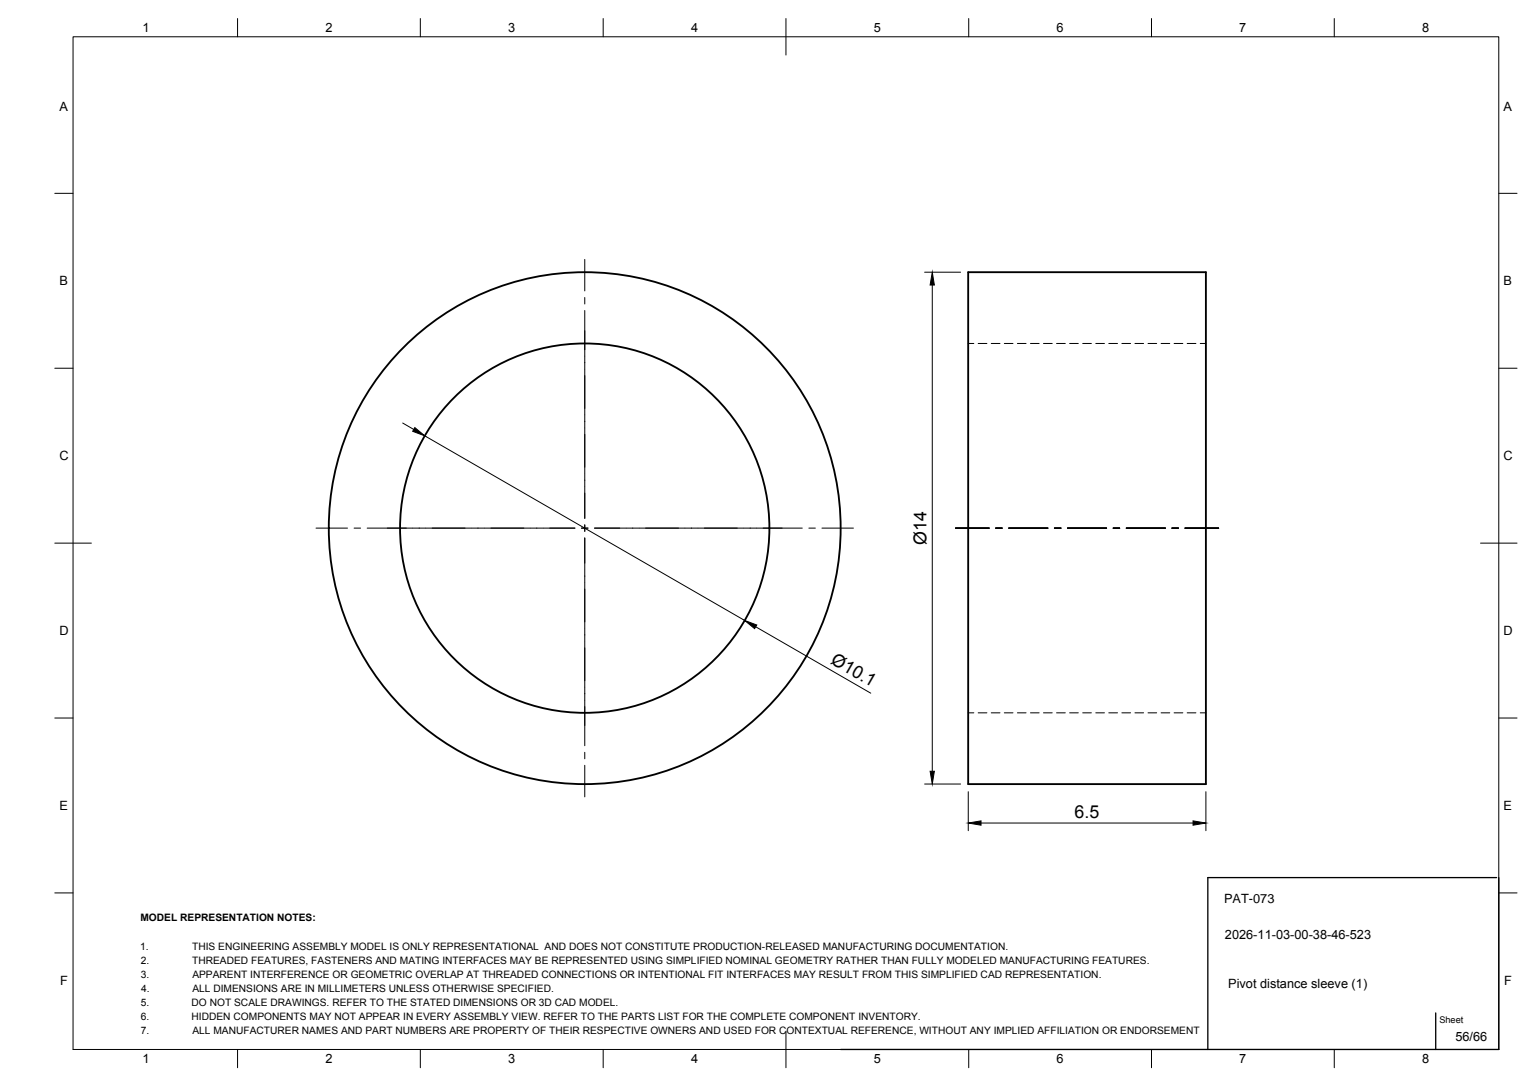
ISO-10303-21;
HEADER;
/* Generated by software containing ST-Developer
 * from STEP Tools, Inc. (www.steptools.com) 
 */

FILE_DESCRIPTION(
/* description */ ('Manual piston pump'),
/* implementation_level */ '2;1');

FILE_NAME(
/* name */ 'Pivot distance sleeve (1).step',
/* time_stamp */ '2026-11-02T16:54:23-08:00',
/* author */ (''),
/* organization */ (''),
/* preprocessor_version */ 'ST-DEVELOPER v20.2',
/* originating_system */ 'Autodesk Translation Framework v15.17.0.0',
/* authorisation */ '');

FILE_SCHEMA (('AUTOMOTIVE_DESIGN { 1 0 10303 214 3 1 1 }'));
ENDSEC;

DATA;
#10=MECHANICAL_DESIGN_GEOMETRIC_PRESENTATION_REPRESENTATION('',(#746),#19043);
#612=SHAPE_REPRESENTATION_RELATIONSHIP('SRR','None',#19362,#675);
#675=ADVANCED_BREP_SHAPE_REPRESENTATION('',(#814),#19029);
#746=STYLED_ITEM('',(#19664),#814);
#814=MANIFOLD_SOLID_BREP('Body1',#9534);
#1022=FACE_BOUND('',#2543,.T.);
#1023=FACE_BOUND('',#2545,.T.);
#1259=CYLINDRICAL_SURFACE('',#11283,0.505000000000001);
#1260=CYLINDRICAL_SURFACE('',#11286,0.699999999999999);
#1770=FACE_OUTER_BOUND('',#2540,.T.);
#1771=FACE_OUTER_BOUND('',#2541,.T.);
#1772=FACE_OUTER_BOUND('',#2542,.T.);
#1773=FACE_OUTER_BOUND('',#2544,.T.);
#2540=EDGE_LOOP('',(#8185,#8186,#8187,#8188));
#2541=EDGE_LOOP('',(#8189,#8190,#8191,#8192));
#2542=EDGE_LOOP('',(#8193));
#2543=EDGE_LOOP('',(#8194));
#2544=EDGE_LOOP('',(#8195));
#2545=EDGE_LOOP('',(#8196));
#3076=CIRCLE('',#11284,0.505000000000001);
#3077=CIRCLE('',#11285,0.505000000000001);
#3078=CIRCLE('',#11287,0.699999999999999);
#3079=CIRCLE('',#11288,0.699999999999999);
#3642=LINE('',#18334,#4246);
#3643=LINE('',#18340,#4247);
#4246=VECTOR('',#14074,0.505000000000001);
#4247=VECTOR('',#14081,0.699999999999999);
#4996=VERTEX_POINT('',#18331);
#4997=VERTEX_POINT('',#18333);
#4998=VERTEX_POINT('',#18337);
#4999=VERTEX_POINT('',#18339);
#6079=EDGE_CURVE('',#4996,#4996,#3076,.T.);
#6080=EDGE_CURVE('',#4996,#4997,#3642,.T.);
#6081=EDGE_CURVE('',#4997,#4997,#3077,.T.);
#6082=EDGE_CURVE('',#4998,#4998,#3078,.T.);
#6083=EDGE_CURVE('',#4998,#4999,#3643,.T.);
#6084=EDGE_CURVE('',#4999,#4999,#3079,.T.);
#8185=ORIENTED_EDGE('',*,*,#6079,.F.);
#8186=ORIENTED_EDGE('',*,*,#6080,.T.);
#8187=ORIENTED_EDGE('',*,*,#6081,.T.);
#8188=ORIENTED_EDGE('',*,*,#6080,.F.);
#8189=ORIENTED_EDGE('',*,*,#6082,.F.);
#8190=ORIENTED_EDGE('',*,*,#6083,.T.);
#8191=ORIENTED_EDGE('',*,*,#6084,.T.);
#8192=ORIENTED_EDGE('',*,*,#6083,.F.);
#8193=ORIENTED_EDGE('',*,*,#6082,.T.);
#8194=ORIENTED_EDGE('',*,*,#6079,.T.);
#8195=ORIENTED_EDGE('',*,*,#6084,.F.);
#8196=ORIENTED_EDGE('',*,*,#6081,.F.);
#8838=PLANE('',#11289);
#8839=PLANE('',#11290);
#9375=ADVANCED_FACE('',(#1770),#1259,.F.);
#9376=ADVANCED_FACE('',(#1771),#1260,.T.);
#9377=ADVANCED_FACE('',(#1772,#1022),#8838,.T.);
#9378=ADVANCED_FACE('',(#1773,#1023),#8839,.F.);
#9534=CLOSED_SHELL('',(#9375,#9376,#9377,#9378));
#11282=AXIS2_PLACEMENT_3D('',#18329,#14068,#14069);
#11283=AXIS2_PLACEMENT_3D('',#18330,#14070,#14071);
#11284=AXIS2_PLACEMENT_3D('',#18332,#14072,#14073);
#11285=AXIS2_PLACEMENT_3D('',#18335,#14075,#14076);
#11286=AXIS2_PLACEMENT_3D('',#18336,#14077,#14078);
#11287=AXIS2_PLACEMENT_3D('',#18338,#14079,#14080);
#11288=AXIS2_PLACEMENT_3D('',#18341,#14082,#14083);
#11289=AXIS2_PLACEMENT_3D('',#18342,#14084,#14085);
#11290=AXIS2_PLACEMENT_3D('',#18343,#14086,#14087);
#14068=DIRECTION('axis',(0.,0.,1.));
#14069=DIRECTION('refdir',(1.,0.,0.));
#14070=DIRECTION('center_axis',(1.,0.,0.));
#14071=DIRECTION('ref_axis',(0.,0.,-1.));
#14072=DIRECTION('center_axis',(-1.,0.,0.));
#14073=DIRECTION('ref_axis',(0.,0.,-1.));
#14074=DIRECTION('',(-1.,0.,0.));
#14075=DIRECTION('center_axis',(-1.,0.,0.));
#14076=DIRECTION('ref_axis',(0.,0.,-1.));
#14077=DIRECTION('center_axis',(1.,0.,0.));
#14078=DIRECTION('ref_axis',(0.,0.,-1.));
#14079=DIRECTION('center_axis',(1.,0.,0.));
#14080=DIRECTION('ref_axis',(0.,0.,-1.));
#14081=DIRECTION('',(-1.,0.,0.));
#14082=DIRECTION('center_axis',(1.,0.,0.));
#14083=DIRECTION('ref_axis',(0.,0.,-1.));
#14084=DIRECTION('center_axis',(1.,0.,0.));
#14085=DIRECTION('ref_axis',(0.,0.,-1.));
#14086=DIRECTION('center_axis',(1.,0.,0.));
#14087=DIRECTION('ref_axis',(0.,0.,-1.));
#18329=CARTESIAN_POINT('',(0.,0.,0.));
#18330=CARTESIAN_POINT('Origin',(-2.05,-4.,10.));
#18331=CARTESIAN_POINT('',(-1.4,-4.,10.505));
#18332=CARTESIAN_POINT('Origin',(-1.4,-4.,10.));
#18333=CARTESIAN_POINT('',(-2.05,-4.,10.505));
#18334=CARTESIAN_POINT('',(-2.05,-4.,10.505));
#18335=CARTESIAN_POINT('Origin',(-2.05,-4.,10.));
#18336=CARTESIAN_POINT('Origin',(-2.05,-4.,10.));
#18337=CARTESIAN_POINT('',(-1.4,-4.,10.7));
#18338=CARTESIAN_POINT('Origin',(-1.4,-4.,10.));
#18339=CARTESIAN_POINT('',(-2.05,-4.,10.7));
#18340=CARTESIAN_POINT('',(-2.05,-4.,10.7));
#18341=CARTESIAN_POINT('Origin',(-2.05,-4.,10.));
#18342=CARTESIAN_POINT('Origin',(-1.4,-4.,10.));
#18343=CARTESIAN_POINT('Origin',(-2.05,-4.,10.));
#18958=UNCERTAINTY_MEASURE_WITH_UNIT(LENGTH_MEASURE(0.001),#19044,
'DISTANCE_ACCURACY_VALUE',
'Maximum model space distance between geometric entities at asserted c
onnectivities');
#18972=UNCERTAINTY_MEASURE_WITH_UNIT(LENGTH_MEASURE(0.001),#19044,
'DISTANCE_ACCURACY_VALUE',
'Maximum model space distance between geometric entities at asserted c
onnectivities');
#19029=(
GEOMETRIC_REPRESENTATION_CONTEXT(3)
GLOBAL_UNCERTAINTY_ASSIGNED_CONTEXT((#18958))
GLOBAL_UNIT_ASSIGNED_CONTEXT((#19044,#19046,#19047))
REPRESENTATION_CONTEXT('','3D')
);
#19043=(
GEOMETRIC_REPRESENTATION_CONTEXT(3)
GLOBAL_UNCERTAINTY_ASSIGNED_CONTEXT((#18972))
GLOBAL_UNIT_ASSIGNED_CONTEXT((#19044,#19046,#19047))
REPRESENTATION_CONTEXT('','3D')
);
#19044=(
LENGTH_UNIT()
NAMED_UNIT(*)
SI_UNIT(.CENTI.,.METRE.)
);
#19046=(
NAMED_UNIT(*)
PLANE_ANGLE_UNIT()
SI_UNIT($,.RADIAN.)
);
#19047=(
NAMED_UNIT(*)
SI_UNIT($,.STERADIAN.)
SOLID_ANGLE_UNIT()
);
#19104=SHAPE_DEFINITION_REPRESENTATION(#19261,#19362);
#19261=PRODUCT_DEFINITION_SHAPE('',$,#19433);
#19362=SHAPE_REPRESENTATION('',(#11282),#19029);
#19376=PRODUCT_DEFINITION_CONTEXT('part definition',#19588,'design');
#19433=PRODUCT_DEFINITION('2026-11-03-00-38-46-523',
'Pivot distance sleeve (1)',#19503,#19376);
#19503=PRODUCT_DEFINITION_FORMATION('',$,#19646);
#19588=APPLICATION_CONTEXT(
'Core Data for Automotive Mechanical Design Process');
#19589=PRODUCT_CONTEXT('part definition',#19588,'mechanical');
#19646=PRODUCT('2026-11-03-00-38-46-523','Pivot distance sleeve (1)',
'Pivot distance sleeve',(#19589));
#19664=PRESENTATION_STYLE_ASSIGNMENT((#19670));
#19670=SURFACE_STYLE_USAGE(.BOTH.,#19676);
#19676=SURFACE_SIDE_STYLE('',(#19682));
#19682=SURFACE_STYLE_FILL_AREA(#19688);
#19688=FILL_AREA_STYLE('CAD Library Painted - Steel gray',(#19694));
#19694=FILL_AREA_STYLE_COLOUR('CAD Library Painted - Steel gray',#19700);
#19700=COLOUR_RGB('CAD Library Painted - Steel gray',0.592156862745098,
0.631372549019608,0.67843137254902);
ENDSEC;
END-ISO-10303-21;
